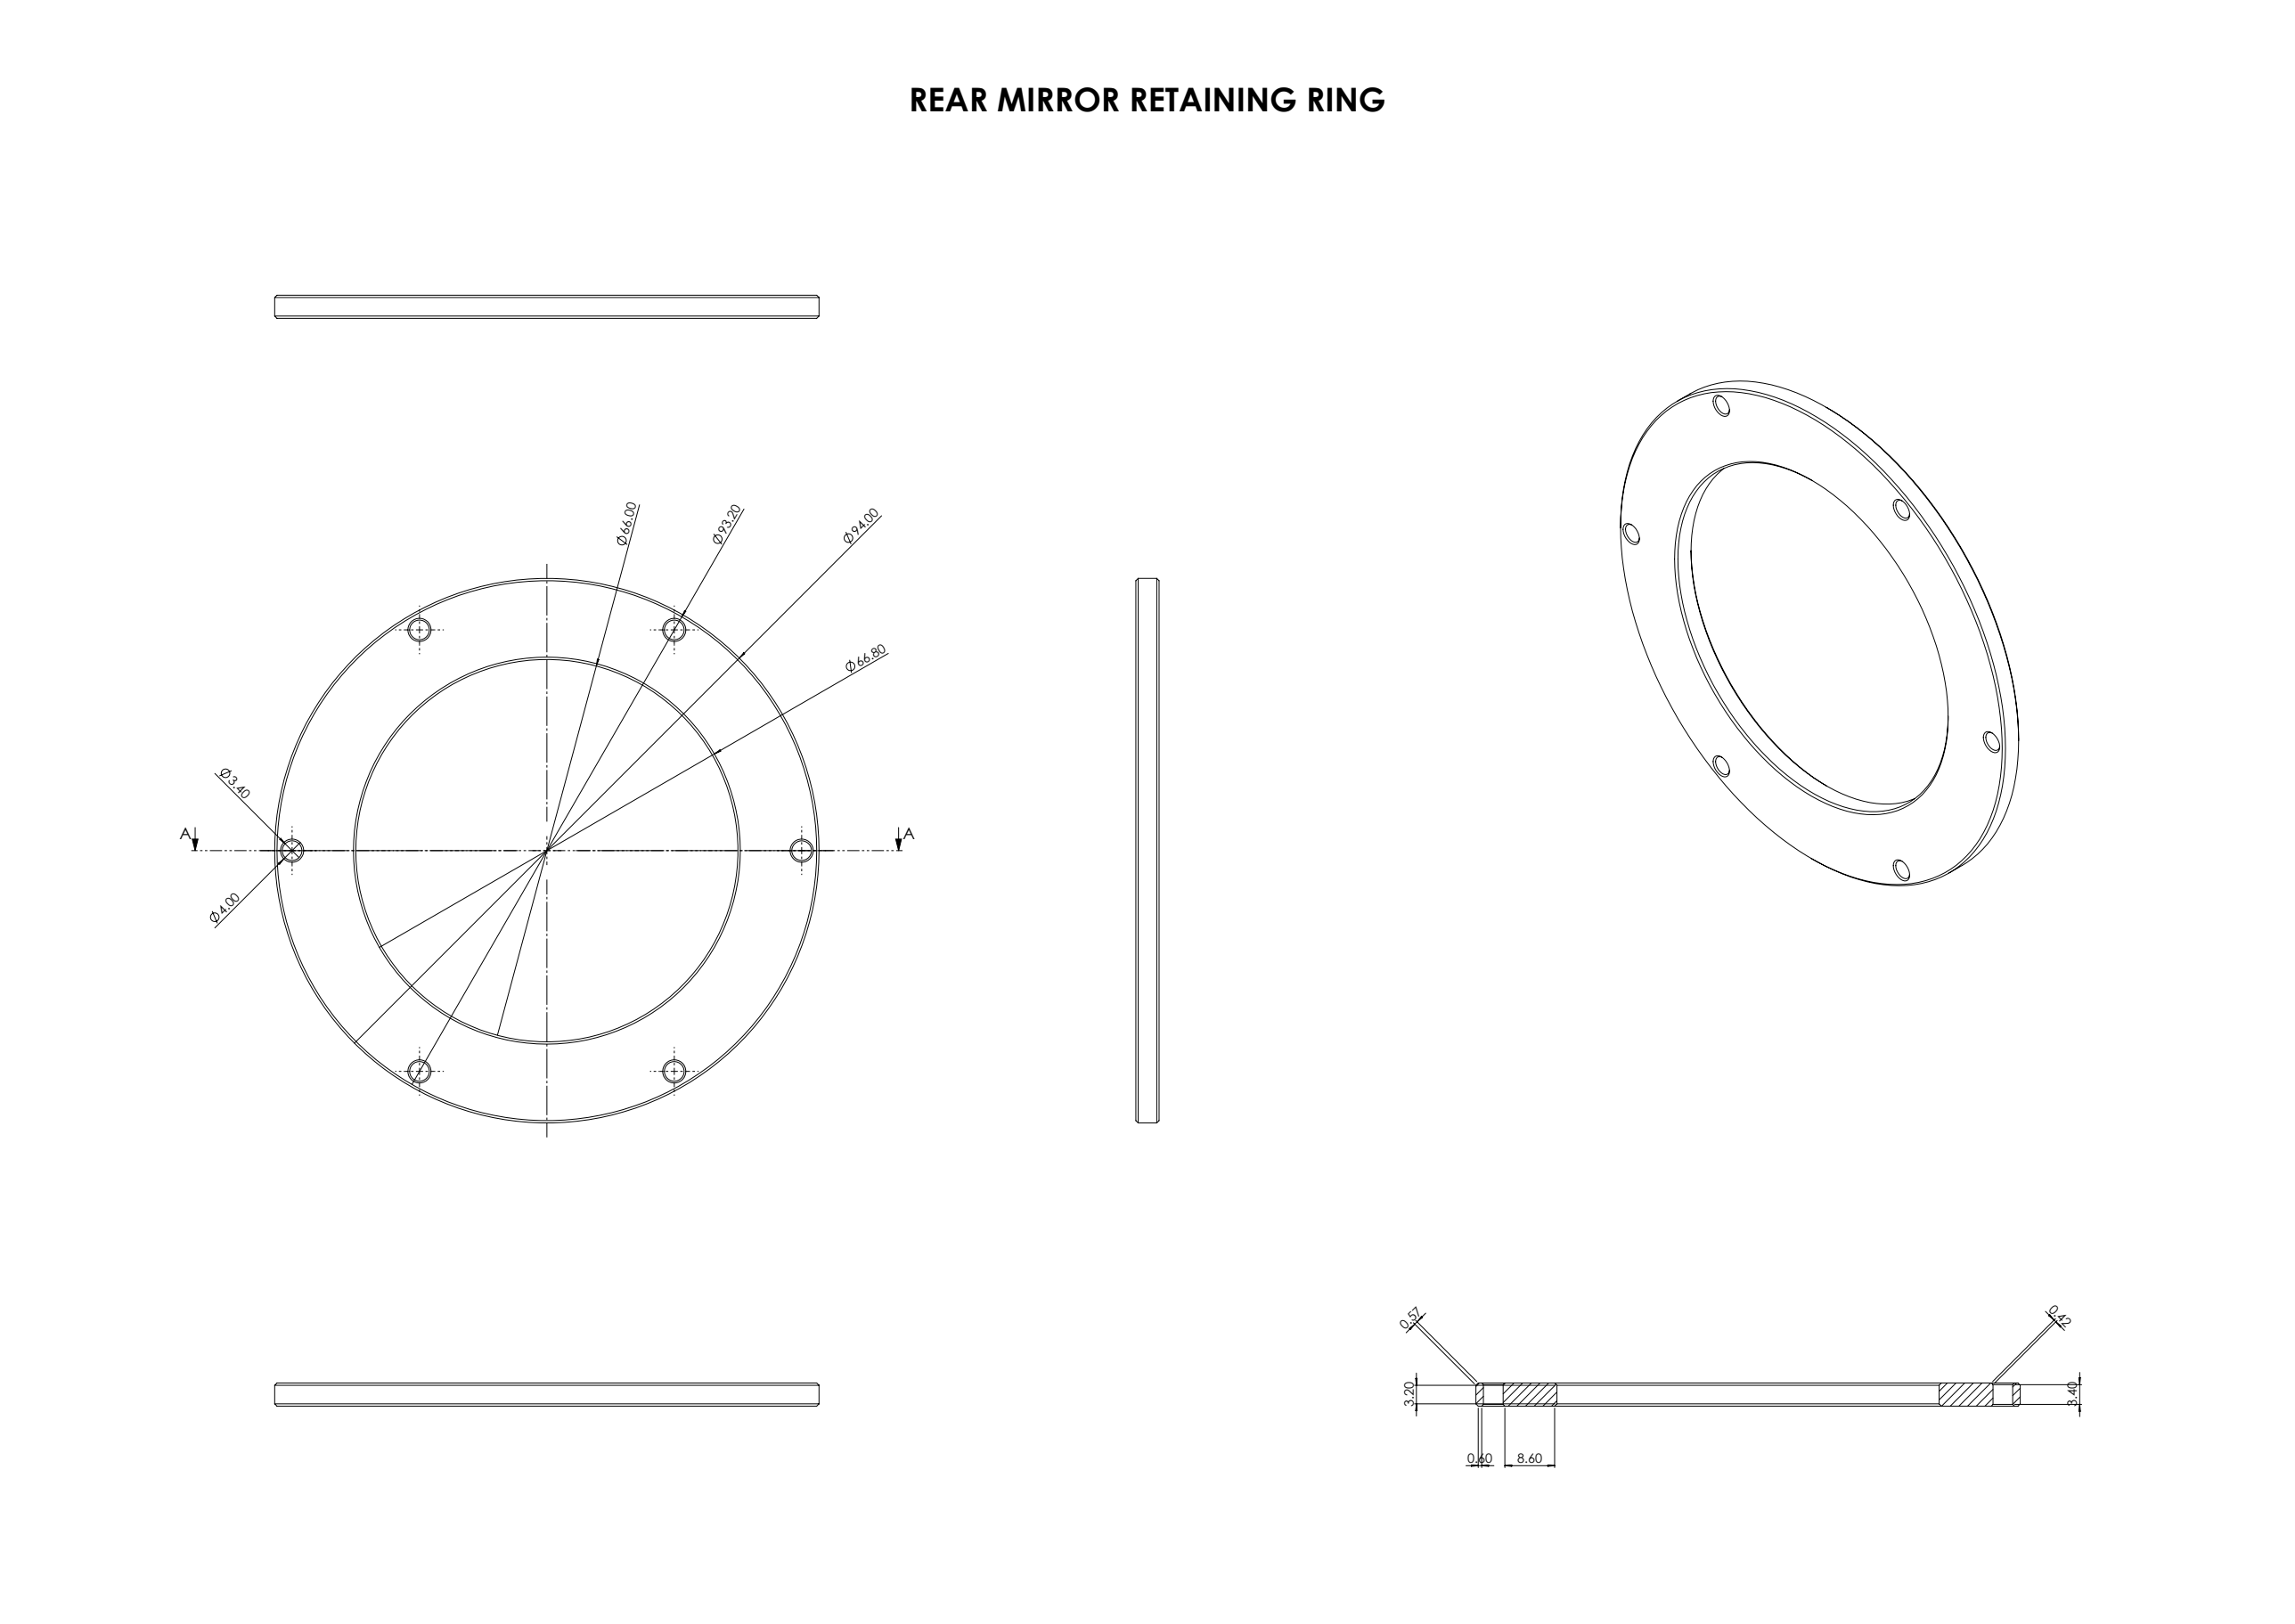
ISO-10303-21;
HEADER;
/* Generated by software containing ST-Developer
 * from STEP Tools, Inc. (www.steptools.com) 
 */

FILE_DESCRIPTION(
/* description */ (''),
/* implementation_level */ '2;1');

FILE_NAME(
/* name */ '12_Rear_Mirror_Retaining_Ring.step',
/* time_stamp */ '2026-10-19T22:59:19-07:00',
/* author */ (''),
/* organization */ (''),
/* preprocessor_version */ 'ST-DEVELOPER v20.2',
/* originating_system */ 'Autodesk Translation Framework v15.15.0.0',
/* authorisation */ '');

FILE_SCHEMA (('AUTOMOTIVE_DESIGN { 1 0 10303 214 3 1 1 }'));
ENDSEC;

DATA;
#10=MECHANICAL_DESIGN_GEOMETRIC_PRESENTATION_REPRESENTATION('',(#915),#53650);
#883=SHAPE_REPRESENTATION_RELATIONSHIP('SRR','None',#53728,#899);
#899=ADVANCED_BREP_SHAPE_REPRESENTATION('',(#931),#53638);
#915=STYLED_ITEM('',(#53944),#931);
#931=MANIFOLD_SOLID_BREP('Retaining Ring',#23307);
#992=CYLINDRICAL_SURFACE('',#24043,0.17);
#993=CYLINDRICAL_SURFACE('',#24066,0.17);
#994=CYLINDRICAL_SURFACE('',#24072,0.17);
#995=CYLINDRICAL_SURFACE('',#24078,0.170000000000001);
#996=CYLINDRICAL_SURFACE('',#24084,0.17);
#997=CYLINDRICAL_SURFACE('',#24090,0.17);
#998=CYLINDRICAL_SURFACE('',#24096,4.7);
#999=CYLINDRICAL_SURFACE('',#24103,3.3);
#1331=FACE_BOUND('',#3914,.T.);
#1332=FACE_BOUND('',#3915,.T.);
#1333=FACE_BOUND('',#3916,.T.);
#1334=FACE_BOUND('',#3917,.T.);
#1335=FACE_BOUND('',#3918,.T.);
#1336=FACE_BOUND('',#3919,.T.);
#1337=FACE_BOUND('',#3920,.T.);
#1338=FACE_BOUND('',#3923,.T.);
#1339=FACE_BOUND('',#3924,.T.);
#1340=FACE_BOUND('',#3925,.T.);
#1341=FACE_BOUND('',#3926,.T.);
#1342=FACE_BOUND('',#3927,.T.);
#1343=FACE_BOUND('',#3928,.T.);
#1344=FACE_BOUND('',#3929,.T.);
#1551=PLANE('',#24045);
#1552=PLANE('',#24055);
#2529=FACE_OUTER_BOUND('',#3911,.T.);
#2530=FACE_OUTER_BOUND('',#3912,.T.);
#2531=FACE_OUTER_BOUND('',#3913,.T.);
#2532=FACE_OUTER_BOUND('',#3921,.T.);
#2533=FACE_OUTER_BOUND('',#3922,.T.);
#2534=FACE_OUTER_BOUND('',#3930,.T.);
#2535=FACE_OUTER_BOUND('',#3931,.T.);
#2536=FACE_OUTER_BOUND('',#3932,.T.);
#2537=FACE_OUTER_BOUND('',#3933,.T.);
#2538=FACE_OUTER_BOUND('',#3934,.T.);
#2539=FACE_OUTER_BOUND('',#3935,.T.);
#2540=FACE_OUTER_BOUND('',#3936,.T.);
#2541=FACE_OUTER_BOUND('',#3937,.T.);
#2542=FACE_OUTER_BOUND('',#3938,.T.);
#2543=FACE_OUTER_BOUND('',#3939,.T.);
#2544=FACE_OUTER_BOUND('',#3940,.T.);
#2545=FACE_OUTER_BOUND('',#3941,.T.);
#2546=FACE_OUTER_BOUND('',#3942,.T.);
#2547=FACE_OUTER_BOUND('',#3943,.T.);
#2548=FACE_OUTER_BOUND('',#3944,.T.);
#2549=FACE_OUTER_BOUND('',#3945,.T.);
#2550=FACE_OUTER_BOUND('',#3946,.T.);
#2551=FACE_OUTER_BOUND('',#3947,.T.);
#2552=FACE_OUTER_BOUND('',#3948,.T.);
#2553=FACE_OUTER_BOUND('',#3949,.T.);
#2554=FACE_OUTER_BOUND('',#3950,.T.);
#3911=EDGE_LOOP('',(#16315,#16316,#16317,#16318,#16319));
#3912=EDGE_LOOP('',(#16320,#16321,#16322,#16323,#16324));
#3913=EDGE_LOOP('',(#16325));
#3914=EDGE_LOOP('',(#16326));
#3915=EDGE_LOOP('',(#16327));
#3916=EDGE_LOOP('',(#16328));
#3917=EDGE_LOOP('',(#16329));
#3918=EDGE_LOOP('',(#16330));
#3919=EDGE_LOOP('',(#16331));
#3920=EDGE_LOOP('',(#16332));
#3921=EDGE_LOOP('',(#16333,#16334,#16335,#16336));
#3922=EDGE_LOOP('',(#16337));
#3923=EDGE_LOOP('',(#16338));
#3924=EDGE_LOOP('',(#16339));
#3925=EDGE_LOOP('',(#16340));
#3926=EDGE_LOOP('',(#16341));
#3927=EDGE_LOOP('',(#16342));
#3928=EDGE_LOOP('',(#16343));
#3929=EDGE_LOOP('',(#16344));
#3930=EDGE_LOOP('',(#16345,#16346,#16347,#16348,#16349));
#3931=EDGE_LOOP('',(#16350,#16351,#16352,#16353,#16354));
#3932=EDGE_LOOP('',(#16355,#16356,#16357,#16358));
#3933=EDGE_LOOP('',(#16359,#16360,#16361,#16362,#16363));
#3934=EDGE_LOOP('',(#16364,#16365,#16366,#16367,#16368));
#3935=EDGE_LOOP('',(#16369,#16370,#16371,#16372));
#3936=EDGE_LOOP('',(#16373,#16374,#16375,#16376,#16377));
#3937=EDGE_LOOP('',(#16378,#16379,#16380,#16381,#16382));
#3938=EDGE_LOOP('',(#16383,#16384,#16385,#16386));
#3939=EDGE_LOOP('',(#16387,#16388,#16389,#16390,#16391));
#3940=EDGE_LOOP('',(#16392,#16393,#16394,#16395,#16396));
#3941=EDGE_LOOP('',(#16397,#16398,#16399,#16400));
#3942=EDGE_LOOP('',(#16401,#16402,#16403,#16404,#16405));
#3943=EDGE_LOOP('',(#16406,#16407,#16408,#16409,#16410));
#3944=EDGE_LOOP('',(#16411,#16412,#16413,#16414));
#3945=EDGE_LOOP('',(#16415,#16416,#16417,#16418,#16419));
#3946=EDGE_LOOP('',(#16420,#16421,#16422,#16423,#16424,#16425));
#3947=EDGE_LOOP('',(#16426,#16427,#16428,#16429,#16430));
#3948=EDGE_LOOP('',(#16431,#16432,#16433,#16434,#16435));
#3949=EDGE_LOOP('',(#16436,#16437,#16438,#16439,#16440,#16441));
#3950=EDGE_LOOP('',(#16442,#16443,#16444,#16445,#16446));
#5307=CIRCLE('',#24040,0.2);
#5308=CIRCLE('',#24041,0.17);
#5309=CIRCLE('',#24042,0.17);
#5310=CIRCLE('',#24044,0.17);
#5311=CIRCLE('',#24046,4.66);
#5312=CIRCLE('',#24047,0.2);
#5313=CIRCLE('',#24048,0.200000000000001);
#5314=CIRCLE('',#24049,0.2);
#5315=CIRCLE('',#24050,3.34);
#5316=CIRCLE('',#24051,0.2);
#5317=CIRCLE('',#24052,0.2);
#5318=CIRCLE('',#24054,0.2);
#5319=CIRCLE('',#24056,4.66);
#5320=CIRCLE('',#24057,0.2);
#5321=CIRCLE('',#24058,0.200000000000001);
#5322=CIRCLE('',#24059,0.2);
#5323=CIRCLE('',#24060,3.34);
#5324=CIRCLE('',#24061,0.2);
#5325=CIRCLE('',#24062,0.2);
#5326=CIRCLE('',#24064,0.17);
#5327=CIRCLE('',#24065,0.17);
#5328=CIRCLE('',#24067,0.17);
#5329=CIRCLE('',#24070,0.17);
#5330=CIRCLE('',#24071,0.17);
#5331=CIRCLE('',#24073,0.17);
#5332=CIRCLE('',#24076,0.170000000000001);
#5333=CIRCLE('',#24077,0.170000000000001);
#5334=CIRCLE('',#24079,0.170000000000001);
#5335=CIRCLE('',#24082,0.17);
#5336=CIRCLE('',#24083,0.17);
#5337=CIRCLE('',#24085,0.17);
#5338=CIRCLE('',#24088,0.17);
#5339=CIRCLE('',#24089,0.17);
#5340=CIRCLE('',#24091,0.17);
#5341=CIRCLE('',#24094,4.7);
#5342=CIRCLE('',#24095,4.7);
#5343=CIRCLE('',#24097,4.7);
#5344=CIRCLE('',#24098,4.7);
#5345=CIRCLE('',#24101,3.3);
#5346=CIRCLE('',#24102,3.3);
#5347=CIRCLE('',#24104,3.3);
#5348=CIRCLE('',#24105,3.3);
#6232=LINE('',#33103,#8077);
#6233=LINE('',#33110,#8078);
#6234=LINE('',#33129,#8079);
#6235=LINE('',#33147,#8080);
#6236=LINE('',#33154,#8081);
#6237=LINE('',#33156,#8082);
#6238=LINE('',#33159,#8083);
#6239=LINE('',#33166,#8084);
#6240=LINE('',#33168,#8085);
#6241=LINE('',#33171,#8086);
#6242=LINE('',#33178,#8087);
#6243=LINE('',#33180,#8088);
#6244=LINE('',#33183,#8089);
#6245=LINE('',#33190,#8090);
#6246=LINE('',#33192,#8091);
#6247=LINE('',#33195,#8092);
#6248=LINE('',#33202,#8093);
#6249=LINE('',#33204,#8094);
#6250=LINE('',#33207,#8095);
#6251=LINE('',#33213,#8096);
#6252=LINE('',#33218,#8097);
#6253=LINE('',#33221,#8098);
#6254=LINE('',#33230,#8099);
#6255=LINE('',#33232,#8100);
#8077=VECTOR('',#27124,0.185);
#8078=VECTOR('',#27133,0.17);
#8079=VECTOR('',#27154,0.185);
#8080=VECTOR('',#27173,0.185);
#8081=VECTOR('',#27182,0.17);
#8082=VECTOR('',#27185,0.185);
#8083=VECTOR('',#27188,0.185);
#8084=VECTOR('',#27197,0.17);
#8085=VECTOR('',#27200,0.185);
#8086=VECTOR('',#27203,0.185000000000001);
#8087=VECTOR('',#27212,0.170000000000001);
#8088=VECTOR('',#27215,0.185000000000001);
#8089=VECTOR('',#27218,0.185);
#8090=VECTOR('',#27227,0.17);
#8091=VECTOR('',#27230,0.185);
#8092=VECTOR('',#27233,0.185);
#8093=VECTOR('',#27242,0.17);
#8094=VECTOR('',#27245,0.185);
#8095=VECTOR('',#27248,4.68);
#8096=VECTOR('',#27255,4.7);
#8097=VECTOR('',#27262,4.68);
#8098=VECTOR('',#27265,3.32);
#8099=VECTOR('',#27276,3.3);
#8100=VECTOR('',#27279,3.32);
#9903=VERTEX_POINT('',#33100);
#9904=VERTEX_POINT('',#33102);
#9905=VERTEX_POINT('',#33104);
#9906=VERTEX_POINT('',#33108);
#9907=VERTEX_POINT('',#33112);
#9908=VERTEX_POINT('',#33114);
#9909=VERTEX_POINT('',#33116);
#9910=VERTEX_POINT('',#33118);
#9911=VERTEX_POINT('',#33120);
#9912=VERTEX_POINT('',#33122);
#9913=VERTEX_POINT('',#33124);
#9914=VERTEX_POINT('',#33127);
#9915=VERTEX_POINT('',#33131);
#9916=VERTEX_POINT('',#33133);
#9917=VERTEX_POINT('',#33135);
#9918=VERTEX_POINT('',#33137);
#9919=VERTEX_POINT('',#33139);
#9920=VERTEX_POINT('',#33141);
#9921=VERTEX_POINT('',#33143);
#9922=VERTEX_POINT('',#33146);
#9923=VERTEX_POINT('',#33148);
#9924=VERTEX_POINT('',#33152);
#9925=VERTEX_POINT('',#33158);
#9926=VERTEX_POINT('',#33160);
#9927=VERTEX_POINT('',#33164);
#9928=VERTEX_POINT('',#33170);
#9929=VERTEX_POINT('',#33172);
#9930=VERTEX_POINT('',#33176);
#9931=VERTEX_POINT('',#33182);
#9932=VERTEX_POINT('',#33184);
#9933=VERTEX_POINT('',#33188);
#9934=VERTEX_POINT('',#33194);
#9935=VERTEX_POINT('',#33196);
#9936=VERTEX_POINT('',#33200);
#9937=VERTEX_POINT('',#33206);
#9938=VERTEX_POINT('',#33208);
#9939=VERTEX_POINT('',#33212);
#9940=VERTEX_POINT('',#33214);
#9941=VERTEX_POINT('',#33220);
#9942=VERTEX_POINT('',#33222);
#9943=VERTEX_POINT('',#33226);
#9944=VERTEX_POINT('',#33227);
#12335=EDGE_CURVE('',#9903,#9903,#5307,.T.);
#12336=EDGE_CURVE('',#9903,#9904,#6232,.T.);
#12337=EDGE_CURVE('',#9904,#9905,#5308,.T.);
#12338=EDGE_CURVE('',#9905,#9904,#5309,.T.);
#12339=EDGE_CURVE('',#9906,#9906,#5310,.T.);
#12340=EDGE_CURVE('',#9906,#9905,#6233,.T.);
#12341=EDGE_CURVE('',#9907,#9907,#5311,.T.);
#12342=EDGE_CURVE('',#9908,#9908,#5312,.T.);
#12343=EDGE_CURVE('',#9909,#9909,#5313,.T.);
#12344=EDGE_CURVE('',#9910,#9910,#5314,.T.);
#12345=EDGE_CURVE('',#9911,#9911,#5315,.T.);
#12346=EDGE_CURVE('',#9912,#9912,#5316,.T.);
#12347=EDGE_CURVE('',#9913,#9913,#5317,.T.);
#12348=EDGE_CURVE('',#9914,#9914,#5318,.T.);
#12349=EDGE_CURVE('',#9914,#9906,#6234,.T.);
#12350=EDGE_CURVE('',#9915,#9915,#5319,.T.);
#12351=EDGE_CURVE('',#9916,#9916,#5320,.T.);
#12352=EDGE_CURVE('',#9917,#9917,#5321,.T.);
#12353=EDGE_CURVE('',#9918,#9918,#5322,.T.);
#12354=EDGE_CURVE('',#9919,#9919,#5323,.T.);
#12355=EDGE_CURVE('',#9920,#9920,#5324,.T.);
#12356=EDGE_CURVE('',#9921,#9921,#5325,.T.);
#12357=EDGE_CURVE('',#9908,#9922,#6235,.T.);
#12358=EDGE_CURVE('',#9922,#9923,#5326,.T.);
#12359=EDGE_CURVE('',#9923,#9922,#5327,.T.);
#12360=EDGE_CURVE('',#9924,#9924,#5328,.T.);
#12361=EDGE_CURVE('',#9924,#9923,#6236,.T.);
#12362=EDGE_CURVE('',#9916,#9924,#6237,.T.);
#12363=EDGE_CURVE('',#9913,#9925,#6238,.T.);
#12364=EDGE_CURVE('',#9925,#9926,#5329,.T.);
#12365=EDGE_CURVE('',#9926,#9925,#5330,.T.);
#12366=EDGE_CURVE('',#9927,#9927,#5331,.T.);
#12367=EDGE_CURVE('',#9927,#9926,#6239,.T.);
#12368=EDGE_CURVE('',#9921,#9927,#6240,.T.);
#12369=EDGE_CURVE('',#9909,#9928,#6241,.T.);
#12370=EDGE_CURVE('',#9928,#9929,#5332,.T.);
#12371=EDGE_CURVE('',#9929,#9928,#5333,.T.);
#12372=EDGE_CURVE('',#9930,#9930,#5334,.T.);
#12373=EDGE_CURVE('',#9930,#9929,#6242,.T.);
#12374=EDGE_CURVE('',#9917,#9930,#6243,.T.);
#12375=EDGE_CURVE('',#9912,#9931,#6244,.T.);
#12376=EDGE_CURVE('',#9931,#9932,#5335,.T.);
#12377=EDGE_CURVE('',#9932,#9931,#5336,.T.);
#12378=EDGE_CURVE('',#9933,#9933,#5337,.T.);
#12379=EDGE_CURVE('',#9933,#9932,#6245,.T.);
#12380=EDGE_CURVE('',#9920,#9933,#6246,.T.);
#12381=EDGE_CURVE('',#9910,#9934,#6247,.T.);
#12382=EDGE_CURVE('',#9934,#9935,#5338,.T.);
#12383=EDGE_CURVE('',#9935,#9934,#5339,.T.);
#12384=EDGE_CURVE('',#9936,#9936,#5340,.T.);
#12385=EDGE_CURVE('',#9936,#9935,#6248,.T.);
#12386=EDGE_CURVE('',#9918,#9936,#6249,.T.);
#12387=EDGE_CURVE('',#9907,#9937,#6250,.T.);
#12388=EDGE_CURVE('',#9937,#9938,#5341,.T.);
#12389=EDGE_CURVE('',#9938,#9937,#5342,.T.);
#12390=EDGE_CURVE('',#9938,#9939,#6251,.T.);
#12391=EDGE_CURVE('',#9940,#9939,#5343,.T.);
#12392=EDGE_CURVE('',#9939,#9940,#5344,.T.);
#12393=EDGE_CURVE('',#9940,#9915,#6252,.T.);
#12394=EDGE_CURVE('',#9919,#9941,#6253,.T.);
#12395=EDGE_CURVE('',#9941,#9942,#5345,.T.);
#12396=EDGE_CURVE('',#9942,#9941,#5346,.T.);
#12397=EDGE_CURVE('',#9943,#9944,#5347,.T.);
#12398=EDGE_CURVE('',#9944,#9943,#5348,.T.);
#12399=EDGE_CURVE('',#9944,#9942,#6254,.T.);
#12400=EDGE_CURVE('',#9943,#9911,#6255,.T.);
#16315=ORIENTED_EDGE('',*,*,#12335,.T.);
#16316=ORIENTED_EDGE('',*,*,#12336,.T.);
#16317=ORIENTED_EDGE('',*,*,#12337,.T.);
#16318=ORIENTED_EDGE('',*,*,#12338,.T.);
#16319=ORIENTED_EDGE('',*,*,#12336,.F.);
#16320=ORIENTED_EDGE('',*,*,#12339,.F.);
#16321=ORIENTED_EDGE('',*,*,#12340,.T.);
#16322=ORIENTED_EDGE('',*,*,#12337,.F.);
#16323=ORIENTED_EDGE('',*,*,#12338,.F.);
#16324=ORIENTED_EDGE('',*,*,#12340,.F.);
#16325=ORIENTED_EDGE('',*,*,#12341,.F.);
#16326=ORIENTED_EDGE('',*,*,#12342,.F.);
#16327=ORIENTED_EDGE('',*,*,#12343,.F.);
#16328=ORIENTED_EDGE('',*,*,#12344,.F.);
#16329=ORIENTED_EDGE('',*,*,#12345,.F.);
#16330=ORIENTED_EDGE('',*,*,#12346,.F.);
#16331=ORIENTED_EDGE('',*,*,#12347,.F.);
#16332=ORIENTED_EDGE('',*,*,#12335,.F.);
#16333=ORIENTED_EDGE('',*,*,#12348,.T.);
#16334=ORIENTED_EDGE('',*,*,#12349,.T.);
#16335=ORIENTED_EDGE('',*,*,#12339,.T.);
#16336=ORIENTED_EDGE('',*,*,#12349,.F.);
#16337=ORIENTED_EDGE('',*,*,#12350,.F.);
#16338=ORIENTED_EDGE('',*,*,#12351,.F.);
#16339=ORIENTED_EDGE('',*,*,#12352,.F.);
#16340=ORIENTED_EDGE('',*,*,#12353,.F.);
#16341=ORIENTED_EDGE('',*,*,#12354,.F.);
#16342=ORIENTED_EDGE('',*,*,#12355,.F.);
#16343=ORIENTED_EDGE('',*,*,#12356,.F.);
#16344=ORIENTED_EDGE('',*,*,#12348,.F.);
#16345=ORIENTED_EDGE('',*,*,#12342,.T.);
#16346=ORIENTED_EDGE('',*,*,#12357,.T.);
#16347=ORIENTED_EDGE('',*,*,#12358,.T.);
#16348=ORIENTED_EDGE('',*,*,#12359,.T.);
#16349=ORIENTED_EDGE('',*,*,#12357,.F.);
#16350=ORIENTED_EDGE('',*,*,#12360,.F.);
#16351=ORIENTED_EDGE('',*,*,#12361,.T.);
#16352=ORIENTED_EDGE('',*,*,#12358,.F.);
#16353=ORIENTED_EDGE('',*,*,#12359,.F.);
#16354=ORIENTED_EDGE('',*,*,#12361,.F.);
#16355=ORIENTED_EDGE('',*,*,#12351,.T.);
#16356=ORIENTED_EDGE('',*,*,#12362,.T.);
#16357=ORIENTED_EDGE('',*,*,#12360,.T.);
#16358=ORIENTED_EDGE('',*,*,#12362,.F.);
#16359=ORIENTED_EDGE('',*,*,#12347,.T.);
#16360=ORIENTED_EDGE('',*,*,#12363,.T.);
#16361=ORIENTED_EDGE('',*,*,#12364,.T.);
#16362=ORIENTED_EDGE('',*,*,#12365,.T.);
#16363=ORIENTED_EDGE('',*,*,#12363,.F.);
#16364=ORIENTED_EDGE('',*,*,#12366,.F.);
#16365=ORIENTED_EDGE('',*,*,#12367,.T.);
#16366=ORIENTED_EDGE('',*,*,#12364,.F.);
#16367=ORIENTED_EDGE('',*,*,#12365,.F.);
#16368=ORIENTED_EDGE('',*,*,#12367,.F.);
#16369=ORIENTED_EDGE('',*,*,#12356,.T.);
#16370=ORIENTED_EDGE('',*,*,#12368,.T.);
#16371=ORIENTED_EDGE('',*,*,#12366,.T.);
#16372=ORIENTED_EDGE('',*,*,#12368,.F.);
#16373=ORIENTED_EDGE('',*,*,#12343,.T.);
#16374=ORIENTED_EDGE('',*,*,#12369,.T.);
#16375=ORIENTED_EDGE('',*,*,#12370,.T.);
#16376=ORIENTED_EDGE('',*,*,#12371,.T.);
#16377=ORIENTED_EDGE('',*,*,#12369,.F.);
#16378=ORIENTED_EDGE('',*,*,#12372,.F.);
#16379=ORIENTED_EDGE('',*,*,#12373,.T.);
#16380=ORIENTED_EDGE('',*,*,#12370,.F.);
#16381=ORIENTED_EDGE('',*,*,#12371,.F.);
#16382=ORIENTED_EDGE('',*,*,#12373,.F.);
#16383=ORIENTED_EDGE('',*,*,#12352,.T.);
#16384=ORIENTED_EDGE('',*,*,#12374,.T.);
#16385=ORIENTED_EDGE('',*,*,#12372,.T.);
#16386=ORIENTED_EDGE('',*,*,#12374,.F.);
#16387=ORIENTED_EDGE('',*,*,#12346,.T.);
#16388=ORIENTED_EDGE('',*,*,#12375,.T.);
#16389=ORIENTED_EDGE('',*,*,#12376,.T.);
#16390=ORIENTED_EDGE('',*,*,#12377,.T.);
#16391=ORIENTED_EDGE('',*,*,#12375,.F.);
#16392=ORIENTED_EDGE('',*,*,#12378,.F.);
#16393=ORIENTED_EDGE('',*,*,#12379,.T.);
#16394=ORIENTED_EDGE('',*,*,#12376,.F.);
#16395=ORIENTED_EDGE('',*,*,#12377,.F.);
#16396=ORIENTED_EDGE('',*,*,#12379,.F.);
#16397=ORIENTED_EDGE('',*,*,#12355,.T.);
#16398=ORIENTED_EDGE('',*,*,#12380,.T.);
#16399=ORIENTED_EDGE('',*,*,#12378,.T.);
#16400=ORIENTED_EDGE('',*,*,#12380,.F.);
#16401=ORIENTED_EDGE('',*,*,#12344,.T.);
#16402=ORIENTED_EDGE('',*,*,#12381,.T.);
#16403=ORIENTED_EDGE('',*,*,#12382,.T.);
#16404=ORIENTED_EDGE('',*,*,#12383,.T.);
#16405=ORIENTED_EDGE('',*,*,#12381,.F.);
#16406=ORIENTED_EDGE('',*,*,#12384,.F.);
#16407=ORIENTED_EDGE('',*,*,#12385,.T.);
#16408=ORIENTED_EDGE('',*,*,#12382,.F.);
#16409=ORIENTED_EDGE('',*,*,#12383,.F.);
#16410=ORIENTED_EDGE('',*,*,#12385,.F.);
#16411=ORIENTED_EDGE('',*,*,#12353,.T.);
#16412=ORIENTED_EDGE('',*,*,#12386,.T.);
#16413=ORIENTED_EDGE('',*,*,#12384,.T.);
#16414=ORIENTED_EDGE('',*,*,#12386,.F.);
#16415=ORIENTED_EDGE('',*,*,#12341,.T.);
#16416=ORIENTED_EDGE('',*,*,#12387,.T.);
#16417=ORIENTED_EDGE('',*,*,#12388,.T.);
#16418=ORIENTED_EDGE('',*,*,#12389,.T.);
#16419=ORIENTED_EDGE('',*,*,#12387,.F.);
#16420=ORIENTED_EDGE('',*,*,#12388,.F.);
#16421=ORIENTED_EDGE('',*,*,#12389,.F.);
#16422=ORIENTED_EDGE('',*,*,#12390,.T.);
#16423=ORIENTED_EDGE('',*,*,#12391,.F.);
#16424=ORIENTED_EDGE('',*,*,#12392,.F.);
#16425=ORIENTED_EDGE('',*,*,#12390,.F.);
#16426=ORIENTED_EDGE('',*,*,#12391,.T.);
#16427=ORIENTED_EDGE('',*,*,#12392,.T.);
#16428=ORIENTED_EDGE('',*,*,#12393,.T.);
#16429=ORIENTED_EDGE('',*,*,#12350,.T.);
#16430=ORIENTED_EDGE('',*,*,#12393,.F.);
#16431=ORIENTED_EDGE('',*,*,#12354,.T.);
#16432=ORIENTED_EDGE('',*,*,#12394,.T.);
#16433=ORIENTED_EDGE('',*,*,#12395,.T.);
#16434=ORIENTED_EDGE('',*,*,#12396,.T.);
#16435=ORIENTED_EDGE('',*,*,#12394,.F.);
#16436=ORIENTED_EDGE('',*,*,#12397,.F.);
#16437=ORIENTED_EDGE('',*,*,#12398,.F.);
#16438=ORIENTED_EDGE('',*,*,#12399,.T.);
#16439=ORIENTED_EDGE('',*,*,#12395,.F.);
#16440=ORIENTED_EDGE('',*,*,#12396,.F.);
#16441=ORIENTED_EDGE('',*,*,#12399,.F.);
#16442=ORIENTED_EDGE('',*,*,#12397,.T.);
#16443=ORIENTED_EDGE('',*,*,#12398,.T.);
#16444=ORIENTED_EDGE('',*,*,#12400,.T.);
#16445=ORIENTED_EDGE('',*,*,#12345,.T.);
#16446=ORIENTED_EDGE('',*,*,#12400,.F.);
#21920=CONICAL_SURFACE('',#24039,0.185,0.785398163397452);
#21921=CONICAL_SURFACE('',#24053,0.185,0.785398163397452);
#21922=CONICAL_SURFACE('',#24063,0.185,0.785398163397444);
#21923=CONICAL_SURFACE('',#24068,0.185,0.785398163397445);
#21924=CONICAL_SURFACE('',#24069,0.185,0.785398163397444);
#21925=CONICAL_SURFACE('',#24074,0.185,0.785398163397449);
#21926=CONICAL_SURFACE('',#24075,0.185000000000001,0.785398163397452);
#21927=CONICAL_SURFACE('',#24080,0.185000000000001,0.785398163397452);
#21928=CONICAL_SURFACE('',#24081,0.185,0.785398163397444);
#21929=CONICAL_SURFACE('',#24086,0.185,0.785398163397445);
#21930=CONICAL_SURFACE('',#24087,0.185,0.785398163397444);
#21931=CONICAL_SURFACE('',#24092,0.185,0.785398163397445);
#21932=CONICAL_SURFACE('',#24093,4.68,0.785398163397448);
#21933=CONICAL_SURFACE('',#24099,4.68,0.785398163397449);
#21934=CONICAL_SURFACE('',#24100,3.32,0.785398163397449);
#21935=CONICAL_SURFACE('',#24106,3.32,0.785398163397448);
#22268=ADVANCED_FACE('',(#2529),#21920,.F.);
#22269=ADVANCED_FACE('',(#2530),#992,.F.);
#22270=ADVANCED_FACE('',(#2531,#1331,#1332,#1333,#1334,#1335,#1336,#1337),
#1551,.T.);
#22271=ADVANCED_FACE('',(#2532),#21921,.F.);
#22272=ADVANCED_FACE('',(#2533,#1338,#1339,#1340,#1341,#1342,#1343,#1344),
#1552,.T.);
#22273=ADVANCED_FACE('',(#2534),#21922,.F.);
#22274=ADVANCED_FACE('',(#2535),#993,.F.);
#22275=ADVANCED_FACE('',(#2536),#21923,.F.);
#22276=ADVANCED_FACE('',(#2537),#21924,.F.);
#22277=ADVANCED_FACE('',(#2538),#994,.F.);
#22278=ADVANCED_FACE('',(#2539),#21925,.F.);
#22279=ADVANCED_FACE('',(#2540),#21926,.F.);
#22280=ADVANCED_FACE('',(#2541),#995,.F.);
#22281=ADVANCED_FACE('',(#2542),#21927,.F.);
#22282=ADVANCED_FACE('',(#2543),#21928,.F.);
#22283=ADVANCED_FACE('',(#2544),#996,.F.);
#22284=ADVANCED_FACE('',(#2545),#21929,.F.);
#22285=ADVANCED_FACE('',(#2546),#21930,.F.);
#22286=ADVANCED_FACE('',(#2547),#997,.F.);
#22287=ADVANCED_FACE('',(#2548),#21931,.F.);
#22288=ADVANCED_FACE('',(#2549),#21932,.T.);
#22289=ADVANCED_FACE('',(#2550),#998,.T.);
#22290=ADVANCED_FACE('',(#2551),#21933,.T.);
#22291=ADVANCED_FACE('',(#2552),#21934,.F.);
#22292=ADVANCED_FACE('',(#2553),#999,.F.);
#22293=ADVANCED_FACE('',(#2554),#21935,.F.);
#23307=CLOSED_SHELL('',(#22268,#22269,#22270,#22271,#22272,#22273,#22274,
#22275,#22276,#22277,#22278,#22279,#22280,#22281,#22282,#22283,#22284,#22285,
#22286,#22287,#22288,#22289,#22290,#22291,#22292,#22293));
#24038=AXIS2_PLACEMENT_3D('',#33098,#27118,#27119);
#24039=AXIS2_PLACEMENT_3D('',#33099,#27120,#27121);
#24040=AXIS2_PLACEMENT_3D('',#33101,#27122,#27123);
#24041=AXIS2_PLACEMENT_3D('',#33105,#27125,#27126);
#24042=AXIS2_PLACEMENT_3D('',#33106,#27127,#27128);
#24043=AXIS2_PLACEMENT_3D('',#33107,#27129,#27130);
#24044=AXIS2_PLACEMENT_3D('',#33109,#27131,#27132);
#24045=AXIS2_PLACEMENT_3D('',#33111,#27134,#27135);
#24046=AXIS2_PLACEMENT_3D('',#33113,#27136,#27137);
#24047=AXIS2_PLACEMENT_3D('',#33115,#27138,#27139);
#24048=AXIS2_PLACEMENT_3D('',#33117,#27140,#27141);
#24049=AXIS2_PLACEMENT_3D('',#33119,#27142,#27143);
#24050=AXIS2_PLACEMENT_3D('',#33121,#27144,#27145);
#24051=AXIS2_PLACEMENT_3D('',#33123,#27146,#27147);
#24052=AXIS2_PLACEMENT_3D('',#33125,#27148,#27149);
#24053=AXIS2_PLACEMENT_3D('',#33126,#27150,#27151);
#24054=AXIS2_PLACEMENT_3D('',#33128,#27152,#27153);
#24055=AXIS2_PLACEMENT_3D('',#33130,#27155,#27156);
#24056=AXIS2_PLACEMENT_3D('',#33132,#27157,#27158);
#24057=AXIS2_PLACEMENT_3D('',#33134,#27159,#27160);
#24058=AXIS2_PLACEMENT_3D('',#33136,#27161,#27162);
#24059=AXIS2_PLACEMENT_3D('',#33138,#27163,#27164);
#24060=AXIS2_PLACEMENT_3D('',#33140,#27165,#27166);
#24061=AXIS2_PLACEMENT_3D('',#33142,#27167,#27168);
#24062=AXIS2_PLACEMENT_3D('',#33144,#27169,#27170);
#24063=AXIS2_PLACEMENT_3D('',#33145,#27171,#27172);
#24064=AXIS2_PLACEMENT_3D('',#33149,#27174,#27175);
#24065=AXIS2_PLACEMENT_3D('',#33150,#27176,#27177);
#24066=AXIS2_PLACEMENT_3D('',#33151,#27178,#27179);
#24067=AXIS2_PLACEMENT_3D('',#33153,#27180,#27181);
#24068=AXIS2_PLACEMENT_3D('',#33155,#27183,#27184);
#24069=AXIS2_PLACEMENT_3D('',#33157,#27186,#27187);
#24070=AXIS2_PLACEMENT_3D('',#33161,#27189,#27190);
#24071=AXIS2_PLACEMENT_3D('',#33162,#27191,#27192);
#24072=AXIS2_PLACEMENT_3D('',#33163,#27193,#27194);
#24073=AXIS2_PLACEMENT_3D('',#33165,#27195,#27196);
#24074=AXIS2_PLACEMENT_3D('',#33167,#27198,#27199);
#24075=AXIS2_PLACEMENT_3D('',#33169,#27201,#27202);
#24076=AXIS2_PLACEMENT_3D('',#33173,#27204,#27205);
#24077=AXIS2_PLACEMENT_3D('',#33174,#27206,#27207);
#24078=AXIS2_PLACEMENT_3D('',#33175,#27208,#27209);
#24079=AXIS2_PLACEMENT_3D('',#33177,#27210,#27211);
#24080=AXIS2_PLACEMENT_3D('',#33179,#27213,#27214);
#24081=AXIS2_PLACEMENT_3D('',#33181,#27216,#27217);
#24082=AXIS2_PLACEMENT_3D('',#33185,#27219,#27220);
#24083=AXIS2_PLACEMENT_3D('',#33186,#27221,#27222);
#24084=AXIS2_PLACEMENT_3D('',#33187,#27223,#27224);
#24085=AXIS2_PLACEMENT_3D('',#33189,#27225,#27226);
#24086=AXIS2_PLACEMENT_3D('',#33191,#27228,#27229);
#24087=AXIS2_PLACEMENT_3D('',#33193,#27231,#27232);
#24088=AXIS2_PLACEMENT_3D('',#33197,#27234,#27235);
#24089=AXIS2_PLACEMENT_3D('',#33198,#27236,#27237);
#24090=AXIS2_PLACEMENT_3D('',#33199,#27238,#27239);
#24091=AXIS2_PLACEMENT_3D('',#33201,#27240,#27241);
#24092=AXIS2_PLACEMENT_3D('',#33203,#27243,#27244);
#24093=AXIS2_PLACEMENT_3D('',#33205,#27246,#27247);
#24094=AXIS2_PLACEMENT_3D('',#33209,#27249,#27250);
#24095=AXIS2_PLACEMENT_3D('',#33210,#27251,#27252);
#24096=AXIS2_PLACEMENT_3D('',#33211,#27253,#27254);
#24097=AXIS2_PLACEMENT_3D('',#33215,#27256,#27257);
#24098=AXIS2_PLACEMENT_3D('',#33216,#27258,#27259);
#24099=AXIS2_PLACEMENT_3D('',#33217,#27260,#27261);
#24100=AXIS2_PLACEMENT_3D('',#33219,#27263,#27264);
#24101=AXIS2_PLACEMENT_3D('',#33223,#27266,#27267);
#24102=AXIS2_PLACEMENT_3D('',#33224,#27268,#27269);
#24103=AXIS2_PLACEMENT_3D('',#33225,#27270,#27271);
#24104=AXIS2_PLACEMENT_3D('',#33228,#27272,#27273);
#24105=AXIS2_PLACEMENT_3D('',#33229,#27274,#27275);
#24106=AXIS2_PLACEMENT_3D('',#33231,#27277,#27278);
#27118=DIRECTION('axis',(0.,0.,1.));
#27119=DIRECTION('refdir',(1.,0.,0.));
#27120=DIRECTION('center_axis',(0.,0.,1.));
#27121=DIRECTION('ref_axis',(-1.,0.,0.));
#27122=DIRECTION('center_axis',(0.,0.,1.));
#27123=DIRECTION('ref_axis',(-1.,0.,0.));
#27124=DIRECTION('',(-0.70710678118655,-8.65956056235496E-17,-0.707106781186545));
#27125=DIRECTION('center_axis',(0.,0.,-1.));
#27126=DIRECTION('ref_axis',(-1.,0.,0.));
#27127=DIRECTION('center_axis',(0.,0.,-1.));
#27128=DIRECTION('ref_axis',(-1.,0.,0.));
#27129=DIRECTION('center_axis',(0.,0.,1.));
#27130=DIRECTION('ref_axis',(1.,0.,0.));
#27131=DIRECTION('center_axis',(0.,0.,1.));
#27132=DIRECTION('ref_axis',(1.,0.,0.));
#27133=DIRECTION('',(0.,0.,1.));
#27134=DIRECTION('center_axis',(0.,0.,1.));
#27135=DIRECTION('ref_axis',(1.,0.,0.));
#27136=DIRECTION('center_axis',(0.,0.,-1.));
#27137=DIRECTION('ref_axis',(-1.,0.,0.));
#27138=DIRECTION('center_axis',(0.,0.,1.));
#27139=DIRECTION('ref_axis',(-1.,0.,0.));
#27140=DIRECTION('center_axis',(0.,0.,1.));
#27141=DIRECTION('ref_axis',(-1.,0.,0.));
#27142=DIRECTION('center_axis',(0.,0.,1.));
#27143=DIRECTION('ref_axis',(-1.,0.,0.));
#27144=DIRECTION('center_axis',(0.,0.,1.));
#27145=DIRECTION('ref_axis',(-1.,0.,0.));
#27146=DIRECTION('center_axis',(0.,0.,1.));
#27147=DIRECTION('ref_axis',(-1.,0.,0.));
#27148=DIRECTION('center_axis',(0.,0.,1.));
#27149=DIRECTION('ref_axis',(-1.,0.,0.));
#27150=DIRECTION('center_axis',(0.,0.,-1.));
#27151=DIRECTION('ref_axis',(1.,0.,0.));
#27152=DIRECTION('center_axis',(0.,0.,-1.));
#27153=DIRECTION('ref_axis',(1.,0.,0.));
#27154=DIRECTION('',(0.707106781186551,-8.65956056235497E-17,0.707106781186544));
#27155=DIRECTION('center_axis',(0.,0.,-1.));
#27156=DIRECTION('ref_axis',(-1.,0.,0.));
#27157=DIRECTION('center_axis',(0.,0.,1.));
#27158=DIRECTION('ref_axis',(-1.,0.,0.));
#27159=DIRECTION('center_axis',(0.,0.,-1.));
#27160=DIRECTION('ref_axis',(1.,0.,0.));
#27161=DIRECTION('center_axis',(0.,0.,-1.));
#27162=DIRECTION('ref_axis',(1.,0.,0.));
#27163=DIRECTION('center_axis',(0.,0.,-1.));
#27164=DIRECTION('ref_axis',(1.,0.,0.));
#27165=DIRECTION('center_axis',(0.,0.,-1.));
#27166=DIRECTION('ref_axis',(-1.,0.,0.));
#27167=DIRECTION('center_axis',(0.,0.,-1.));
#27168=DIRECTION('ref_axis',(1.,0.,0.));
#27169=DIRECTION('center_axis',(0.,0.,-1.));
#27170=DIRECTION('ref_axis',(1.,0.,0.));
#27171=DIRECTION('center_axis',(0.,0.,1.));
#27172=DIRECTION('ref_axis',(-1.,0.,0.));
#27173=DIRECTION('',(-0.707106781186545,-8.6595605623549E-17,-0.70710678118655));
#27174=DIRECTION('center_axis',(0.,0.,-1.));
#27175=DIRECTION('ref_axis',(-1.,0.,0.));
#27176=DIRECTION('center_axis',(0.,0.,-1.));
#27177=DIRECTION('ref_axis',(-1.,0.,0.));
#27178=DIRECTION('center_axis',(0.,0.,1.));
#27179=DIRECTION('ref_axis',(1.,0.,0.));
#27180=DIRECTION('center_axis',(0.,0.,1.));
#27181=DIRECTION('ref_axis',(1.,0.,0.));
#27182=DIRECTION('',(0.,0.,1.));
#27183=DIRECTION('center_axis',(0.,0.,-1.));
#27184=DIRECTION('ref_axis',(1.,0.,0.));
#27185=DIRECTION('',(0.707106781186545,-8.65956056235491E-17,0.70710678118655));
#27186=DIRECTION('center_axis',(0.,0.,1.));
#27187=DIRECTION('ref_axis',(-1.,0.,0.));
#27188=DIRECTION('',(-0.707106781186545,-8.6595605623549E-17,-0.70710678118655));
#27189=DIRECTION('center_axis',(0.,0.,-1.));
#27190=DIRECTION('ref_axis',(-1.,0.,0.));
#27191=DIRECTION('center_axis',(0.,0.,-1.));
#27192=DIRECTION('ref_axis',(-1.,0.,0.));
#27193=DIRECTION('center_axis',(0.,0.,1.));
#27194=DIRECTION('ref_axis',(1.,0.,0.));
#27195=DIRECTION('center_axis',(0.,0.,1.));
#27196=DIRECTION('ref_axis',(1.,0.,0.));
#27197=DIRECTION('',(0.,0.,1.));
#27198=DIRECTION('center_axis',(0.,0.,-1.));
#27199=DIRECTION('ref_axis',(1.,0.,0.));
#27200=DIRECTION('',(0.707106781186548,-8.65956056235494E-17,0.707106781186547));
#27201=DIRECTION('center_axis',(0.,0.,1.));
#27202=DIRECTION('ref_axis',(-1.,0.,0.));
#27203=DIRECTION('',(-0.70710678118655,-8.65956056235496E-17,-0.707106781186545));
#27204=DIRECTION('center_axis',(0.,0.,-1.));
#27205=DIRECTION('ref_axis',(-1.,0.,0.));
#27206=DIRECTION('center_axis',(0.,0.,-1.));
#27207=DIRECTION('ref_axis',(-1.,0.,0.));
#27208=DIRECTION('center_axis',(0.,0.,1.));
#27209=DIRECTION('ref_axis',(1.,0.,0.));
#27210=DIRECTION('center_axis',(0.,0.,1.));
#27211=DIRECTION('ref_axis',(1.,0.,0.));
#27212=DIRECTION('',(0.,0.,1.));
#27213=DIRECTION('center_axis',(0.,0.,-1.));
#27214=DIRECTION('ref_axis',(1.,0.,0.));
#27215=DIRECTION('',(0.70710678118655,-8.65956056235497E-17,0.707106781186545));
#27216=DIRECTION('center_axis',(0.,0.,1.));
#27217=DIRECTION('ref_axis',(-1.,0.,0.));
#27218=DIRECTION('',(-0.707106781186545,-8.6595605623549E-17,-0.70710678118655));
#27219=DIRECTION('center_axis',(0.,0.,-1.));
#27220=DIRECTION('ref_axis',(-1.,0.,0.));
#27221=DIRECTION('center_axis',(0.,0.,-1.));
#27222=DIRECTION('ref_axis',(-1.,0.,0.));
#27223=DIRECTION('center_axis',(0.,0.,1.));
#27224=DIRECTION('ref_axis',(1.,0.,0.));
#27225=DIRECTION('center_axis',(0.,0.,1.));
#27226=DIRECTION('ref_axis',(1.,0.,0.));
#27227=DIRECTION('',(0.,0.,1.));
#27228=DIRECTION('center_axis',(0.,0.,-1.));
#27229=DIRECTION('ref_axis',(1.,0.,0.));
#27230=DIRECTION('',(0.707106781186545,-8.65956056235491E-17,0.70710678118655));
#27231=DIRECTION('center_axis',(0.,0.,1.));
#27232=DIRECTION('ref_axis',(-1.,0.,0.));
#27233=DIRECTION('',(-0.707106781186545,-8.6595605623549E-17,-0.70710678118655));
#27234=DIRECTION('center_axis',(0.,0.,-1.));
#27235=DIRECTION('ref_axis',(-1.,0.,0.));
#27236=DIRECTION('center_axis',(0.,0.,-1.));
#27237=DIRECTION('ref_axis',(-1.,0.,0.));
#27238=DIRECTION('center_axis',(0.,0.,1.));
#27239=DIRECTION('ref_axis',(1.,0.,0.));
#27240=DIRECTION('center_axis',(0.,0.,1.));
#27241=DIRECTION('ref_axis',(1.,0.,0.));
#27242=DIRECTION('',(0.,0.,1.));
#27243=DIRECTION('center_axis',(0.,0.,-1.));
#27244=DIRECTION('ref_axis',(1.,0.,0.));
#27245=DIRECTION('',(0.707106781186545,-8.65956056235491E-17,0.70710678118655));
#27246=DIRECTION('center_axis',(0.,0.,-1.));
#27247=DIRECTION('ref_axis',(-1.,0.,0.));
#27248=DIRECTION('',(0.707106781186548,8.65956056235493E-17,-0.707106781186548));
#27249=DIRECTION('center_axis',(0.,0.,1.));
#27250=DIRECTION('ref_axis',(-1.,0.,0.));
#27251=DIRECTION('center_axis',(0.,0.,1.));
#27252=DIRECTION('ref_axis',(-1.,0.,0.));
#27253=DIRECTION('center_axis',(0.,0.,1.));
#27254=DIRECTION('ref_axis',(1.,0.,0.));
#27255=DIRECTION('',(0.,0.,-1.));
#27256=DIRECTION('center_axis',(0.,0.,-1.));
#27257=DIRECTION('ref_axis',(-1.,0.,0.));
#27258=DIRECTION('center_axis',(0.,0.,-1.));
#27259=DIRECTION('ref_axis',(-1.,0.,0.));
#27260=DIRECTION('center_axis',(0.,0.,1.));
#27261=DIRECTION('ref_axis',(-1.,0.,0.));
#27262=DIRECTION('',(-0.707106781186548,-8.65956056235494E-17,-0.707106781186547));
#27263=DIRECTION('center_axis',(0.,0.,-1.));
#27264=DIRECTION('ref_axis',(-1.,0.,0.));
#27265=DIRECTION('',(-0.707106781186548,8.65956056235494E-17,0.707106781186547));
#27266=DIRECTION('center_axis',(0.,0.,1.));
#27267=DIRECTION('ref_axis',(-1.,0.,0.));
#27268=DIRECTION('center_axis',(0.,0.,1.));
#27269=DIRECTION('ref_axis',(-1.,0.,0.));
#27270=DIRECTION('center_axis',(0.,0.,1.));
#27271=DIRECTION('ref_axis',(1.,0.,0.));
#27272=DIRECTION('center_axis',(0.,0.,-1.));
#27273=DIRECTION('ref_axis',(-1.,0.,0.));
#27274=DIRECTION('center_axis',(0.,0.,-1.));
#27275=DIRECTION('ref_axis',(-1.,0.,0.));
#27276=DIRECTION('',(0.,0.,-1.));
#27277=DIRECTION('center_axis',(0.,0.,1.));
#27278=DIRECTION('ref_axis',(-1.,0.,0.));
#27279=DIRECTION('',(0.707106781186548,-8.65956056235493E-17,0.707106781186548));
#33098=CARTESIAN_POINT('',(0.,0.,0.));
#33099=CARTESIAN_POINT('Origin',(4.4,0.,0.385));
#33100=CARTESIAN_POINT('',(4.6,2.44929359829471E-17,0.4));
#33101=CARTESIAN_POINT('Origin',(4.4,0.,0.4));
#33102=CARTESIAN_POINT('',(4.57,-2.0818995585505E-17,0.37));
#33103=CARTESIAN_POINT('',(4.585,2.2655965784226E-17,0.385));
#33104=CARTESIAN_POINT('',(4.23,-2.0818995585505E-17,0.37));
#33105=CARTESIAN_POINT('Origin',(4.4,0.,0.37));
#33106=CARTESIAN_POINT('Origin',(4.4,0.,0.37));
#33107=CARTESIAN_POINT('Origin',(4.4,0.,0.175));
#33108=CARTESIAN_POINT('',(4.23,-2.0818995585505E-17,0.03));
#33109=CARTESIAN_POINT('Origin',(4.4,0.,0.03));
#33110=CARTESIAN_POINT('',(4.23,-2.0818995585505E-17,0.175));
#33111=CARTESIAN_POINT('Origin',(3.3,0.,0.4));
#33112=CARTESIAN_POINT('',(4.66,-5.70685408402667E-16,0.4));
#33113=CARTESIAN_POINT('Origin',(0.,0.,0.4));
#33114=CARTESIAN_POINT('',(2.4,3.81051177665153,0.4));
#33115=CARTESIAN_POINT('Origin',(2.2,3.81051177665153,0.4));
#33116=CARTESIAN_POINT('',(-4.2,5.63337527607783E-16,0.4));
#33117=CARTESIAN_POINT('Origin',(-4.4,5.38844591624835E-16,0.4));
#33118=CARTESIAN_POINT('',(2.4,-3.81051177665153,0.4));
#33119=CARTESIAN_POINT('Origin',(2.2,-3.81051177665153,0.4));
#33120=CARTESIAN_POINT('',(3.34,4.09032030915216E-16,0.4));
#33121=CARTESIAN_POINT('Origin',(0.,0.,0.4));
#33122=CARTESIAN_POINT('',(-2.,-3.81051177665153,0.4));
#33123=CARTESIAN_POINT('Origin',(-2.2,-3.81051177665153,0.4));
#33124=CARTESIAN_POINT('',(-2.,3.81051177665153,0.4));
#33125=CARTESIAN_POINT('Origin',(-2.2,3.81051177665153,0.4));
#33126=CARTESIAN_POINT('Origin',(4.4,0.,0.015));
#33127=CARTESIAN_POINT('',(4.2,2.44929359829471E-17,0.));
#33128=CARTESIAN_POINT('Origin',(4.4,0.,0.));
#33129=CARTESIAN_POINT('',(4.215,2.2655965784226E-17,0.015));
#33130=CARTESIAN_POINT('Origin',(4.7,0.,0.));
#33131=CARTESIAN_POINT('',(4.66,5.70685408402667E-16,0.));
#33132=CARTESIAN_POINT('Origin',(0.,0.,0.));
#33133=CARTESIAN_POINT('',(2.,3.81051177665153,0.));
#33134=CARTESIAN_POINT('Origin',(2.2,3.81051177665153,0.));
#33135=CARTESIAN_POINT('',(-4.6,5.63337527607783E-16,0.));
#33136=CARTESIAN_POINT('Origin',(-4.4,5.38844591624835E-16,0.));
#33137=CARTESIAN_POINT('',(2.,-3.81051177665153,0.));
#33138=CARTESIAN_POINT('Origin',(2.2,-3.81051177665153,0.));
#33139=CARTESIAN_POINT('',(3.34,-4.09032030915216E-16,0.));
#33140=CARTESIAN_POINT('Origin',(0.,0.,0.));
#33141=CARTESIAN_POINT('',(-2.4,-3.81051177665153,0.));
#33142=CARTESIAN_POINT('Origin',(-2.2,-3.81051177665153,0.));
#33143=CARTESIAN_POINT('',(-2.4,3.81051177665153,0.));
#33144=CARTESIAN_POINT('Origin',(-2.2,3.81051177665153,0.));
#33145=CARTESIAN_POINT('Origin',(2.2,3.81051177665153,0.385));
#33146=CARTESIAN_POINT('',(2.37,3.81051177665153,0.37));
#33147=CARTESIAN_POINT('',(2.385,3.81051177665153,0.385));
#33148=CARTESIAN_POINT('',(2.03,3.81051177665153,0.37));
#33149=CARTESIAN_POINT('Origin',(2.2,3.81051177665153,0.37));
#33150=CARTESIAN_POINT('Origin',(2.2,3.81051177665153,0.37));
#33151=CARTESIAN_POINT('Origin',(2.2,3.81051177665153,0.175));
#33152=CARTESIAN_POINT('',(2.03,3.81051177665153,0.03));
#33153=CARTESIAN_POINT('Origin',(2.2,3.81051177665153,0.03));
#33154=CARTESIAN_POINT('',(2.03,3.81051177665153,0.175));
#33155=CARTESIAN_POINT('Origin',(2.2,3.81051177665153,0.015));
#33156=CARTESIAN_POINT('',(2.015,3.81051177665153,0.015));
#33157=CARTESIAN_POINT('Origin',(-2.2,3.81051177665153,0.385));
#33158=CARTESIAN_POINT('',(-2.03,3.81051177665153,0.37));
#33159=CARTESIAN_POINT('',(-2.015,3.81051177665153,0.385));
#33160=CARTESIAN_POINT('',(-2.37,3.81051177665153,0.37));
#33161=CARTESIAN_POINT('Origin',(-2.2,3.81051177665153,0.37));
#33162=CARTESIAN_POINT('Origin',(-2.2,3.81051177665153,0.37));
#33163=CARTESIAN_POINT('Origin',(-2.2,3.81051177665153,0.175));
#33164=CARTESIAN_POINT('',(-2.37,3.81051177665153,0.03));
#33165=CARTESIAN_POINT('Origin',(-2.2,3.81051177665153,0.03));
#33166=CARTESIAN_POINT('',(-2.37,3.81051177665153,0.175));
#33167=CARTESIAN_POINT('Origin',(-2.2,3.81051177665153,0.015));
#33168=CARTESIAN_POINT('',(-2.385,3.81051177665153,0.015));
#33169=CARTESIAN_POINT('Origin',(-4.4,5.38844591624835E-16,0.385));
#33170=CARTESIAN_POINT('',(-4.23,5.1802559603933E-16,0.37));
#33171=CARTESIAN_POINT('',(-4.215,5.61500557409062E-16,0.385));
#33172=CARTESIAN_POINT('',(-4.57,5.1802559603933E-16,0.37));
#33173=CARTESIAN_POINT('Origin',(-4.4,5.38844591624835E-16,0.37));
#33174=CARTESIAN_POINT('Origin',(-4.4,5.38844591624835E-16,0.37));
#33175=CARTESIAN_POINT('Origin',(-4.4,5.38844591624835E-16,0.175));
#33176=CARTESIAN_POINT('',(-4.57,5.1802559603933E-16,0.03));
#33177=CARTESIAN_POINT('Origin',(-4.4,5.38844591624835E-16,0.03));
#33178=CARTESIAN_POINT('',(-4.57,5.1802559603933E-16,0.175));
#33179=CARTESIAN_POINT('Origin',(-4.4,5.38844591624835E-16,0.015));
#33180=CARTESIAN_POINT('',(-4.585,5.61500557409062E-16,0.015));
#33181=CARTESIAN_POINT('Origin',(-2.2,-3.81051177665153,0.385));
#33182=CARTESIAN_POINT('',(-2.03,-3.81051177665153,0.37));
#33183=CARTESIAN_POINT('',(-2.015,-3.81051177665153,0.385));
#33184=CARTESIAN_POINT('',(-2.37,-3.81051177665153,0.37));
#33185=CARTESIAN_POINT('Origin',(-2.2,-3.81051177665153,0.37));
#33186=CARTESIAN_POINT('Origin',(-2.2,-3.81051177665153,0.37));
#33187=CARTESIAN_POINT('Origin',(-2.2,-3.81051177665153,0.175));
#33188=CARTESIAN_POINT('',(-2.37,-3.81051177665153,0.03));
#33189=CARTESIAN_POINT('Origin',(-2.2,-3.81051177665153,0.03));
#33190=CARTESIAN_POINT('',(-2.37,-3.81051177665153,0.175));
#33191=CARTESIAN_POINT('Origin',(-2.2,-3.81051177665153,0.015));
#33192=CARTESIAN_POINT('',(-2.385,-3.81051177665153,0.015));
#33193=CARTESIAN_POINT('Origin',(2.2,-3.81051177665153,0.385));
#33194=CARTESIAN_POINT('',(2.37,-3.81051177665153,0.37));
#33195=CARTESIAN_POINT('',(2.385,-3.81051177665153,0.385));
#33196=CARTESIAN_POINT('',(2.03,-3.81051177665153,0.37));
#33197=CARTESIAN_POINT('Origin',(2.2,-3.81051177665153,0.37));
#33198=CARTESIAN_POINT('Origin',(2.2,-3.81051177665153,0.37));
#33199=CARTESIAN_POINT('Origin',(2.2,-3.81051177665153,0.175));
#33200=CARTESIAN_POINT('',(2.03,-3.81051177665153,0.03));
#33201=CARTESIAN_POINT('Origin',(2.2,-3.81051177665153,0.03));
#33202=CARTESIAN_POINT('',(2.03,-3.81051177665153,0.175));
#33203=CARTESIAN_POINT('Origin',(2.2,-3.81051177665153,0.015));
#33204=CARTESIAN_POINT('',(2.015,-3.81051177665153,0.015));
#33205=CARTESIAN_POINT('Origin',(0.,0.,0.38));
#33206=CARTESIAN_POINT('',(4.7,5.75583995599256E-16,0.36));
#33207=CARTESIAN_POINT('',(4.68,5.73134702000961E-16,0.38));
#33208=CARTESIAN_POINT('',(-4.7,-5.75583995599256E-16,0.36));
#33209=CARTESIAN_POINT('Origin',(0.,0.,0.36));
#33210=CARTESIAN_POINT('Origin',(0.,0.,0.36));
#33211=CARTESIAN_POINT('Origin',(0.,0.,0.2));
#33212=CARTESIAN_POINT('',(-4.7,-5.75583995599256E-16,0.04));
#33213=CARTESIAN_POINT('',(-4.7,-5.75583995599256E-16,0.2));
#33214=CARTESIAN_POINT('',(4.7,-5.75583995599256E-16,0.04));
#33215=CARTESIAN_POINT('Origin',(0.,0.,0.04));
#33216=CARTESIAN_POINT('Origin',(0.,0.,0.04));
#33217=CARTESIAN_POINT('Origin',(0.,0.,0.02));
#33218=CARTESIAN_POINT('',(4.68,5.73134702000961E-16,0.02));
#33219=CARTESIAN_POINT('Origin',(0.,0.,0.02));
#33220=CARTESIAN_POINT('',(3.3,4.04133443718627E-16,0.04));
#33221=CARTESIAN_POINT('',(3.32,-4.06582737316921E-16,0.02));
#33222=CARTESIAN_POINT('',(-3.3,-4.04133443718627E-16,0.04));
#33223=CARTESIAN_POINT('Origin',(0.,0.,0.04));
#33224=CARTESIAN_POINT('Origin',(0.,0.,0.04));
#33225=CARTESIAN_POINT('Origin',(0.,0.,0.2));
#33226=CARTESIAN_POINT('',(3.3,-4.04133443718627E-16,0.36));
#33227=CARTESIAN_POINT('',(-3.3,-4.04133443718627E-16,0.36));
#33228=CARTESIAN_POINT('Origin',(0.,0.,0.36));
#33229=CARTESIAN_POINT('Origin',(0.,0.,0.36));
#33230=CARTESIAN_POINT('',(-3.3,-4.04133443718627E-16,0.2));
#33231=CARTESIAN_POINT('Origin',(0.,0.,0.38));
#33232=CARTESIAN_POINT('',(3.32,-4.06582737316921E-16,0.38));
#53620=UNCERTAINTY_MEASURE_WITH_UNIT(LENGTH_MEASURE(0.001),#53651,
'DISTANCE_ACCURACY_VALUE',
'Maximum model space distance between geometric entities at asserted c
onnectivities');
#53632=UNCERTAINTY_MEASURE_WITH_UNIT(LENGTH_MEASURE(0.001),#53651,
'DISTANCE_ACCURACY_VALUE',
'Maximum model space distance between geometric entities at asserted c
onnectivities');
#53638=(
GEOMETRIC_REPRESENTATION_CONTEXT(3)
GLOBAL_UNCERTAINTY_ASSIGNED_CONTEXT((#53620))
GLOBAL_UNIT_ASSIGNED_CONTEXT((#53651,#53653,#53654))
REPRESENTATION_CONTEXT('','3D')
);
#53650=(
GEOMETRIC_REPRESENTATION_CONTEXT(3)
GLOBAL_UNCERTAINTY_ASSIGNED_CONTEXT((#53632))
GLOBAL_UNIT_ASSIGNED_CONTEXT((#53651,#53653,#53654))
REPRESENTATION_CONTEXT('','3D')
);
#53651=(
LENGTH_UNIT()
NAMED_UNIT(*)
SI_UNIT(.CENTI.,.METRE.)
);
#53653=(
NAMED_UNIT(*)
PLANE_ANGLE_UNIT()
SI_UNIT($,.RADIAN.)
);
#53654=(
NAMED_UNIT(*)
SI_UNIT($,.STERADIAN.)
SOLID_ANGLE_UNIT()
);
#53660=SHAPE_DEFINITION_REPRESENTATION(#53677,#53728);
#53677=PRODUCT_DEFINITION_SHAPE('',$,#53746);
#53728=SHAPE_REPRESENTATION('',(#24038),#53638);
#53740=PRODUCT_DEFINITION_CONTEXT('part definition',#53793,'design');
#53746=PRODUCT_DEFINITION('2026-10-18-22-44-50-492',
'12_Rear_Mirror_Retaining_Ring',#53763,#53740);
#53763=PRODUCT_DEFINITION_FORMATION('',$,#53800);
#53793=APPLICATION_CONTEXT(
'Core Data for Automotive Mechanical Design Process');
#53794=PRODUCT_CONTEXT('part definition',#53793,'mechanical');
#53800=PRODUCT('2026-10-18-22-44-50-492',
'12_Rear_Mirror_Retaining_Ring',$,(#53794));
#53938=COLOUR_RGB('Light Blue',0.38,0.62,0.78);
#53939=FILL_AREA_STYLE_COLOUR('',#53938);
#53940=FILL_AREA_STYLE('',(#53939));
#53941=SURFACE_STYLE_FILL_AREA(#53940);
#53942=SURFACE_SIDE_STYLE('',(#53941));
#53943=SURFACE_STYLE_USAGE(.BOTH.,#53942);
#53944=PRESENTATION_STYLE_ASSIGNMENT((#53943));
ENDSEC;
END-ISO-10303-21;
